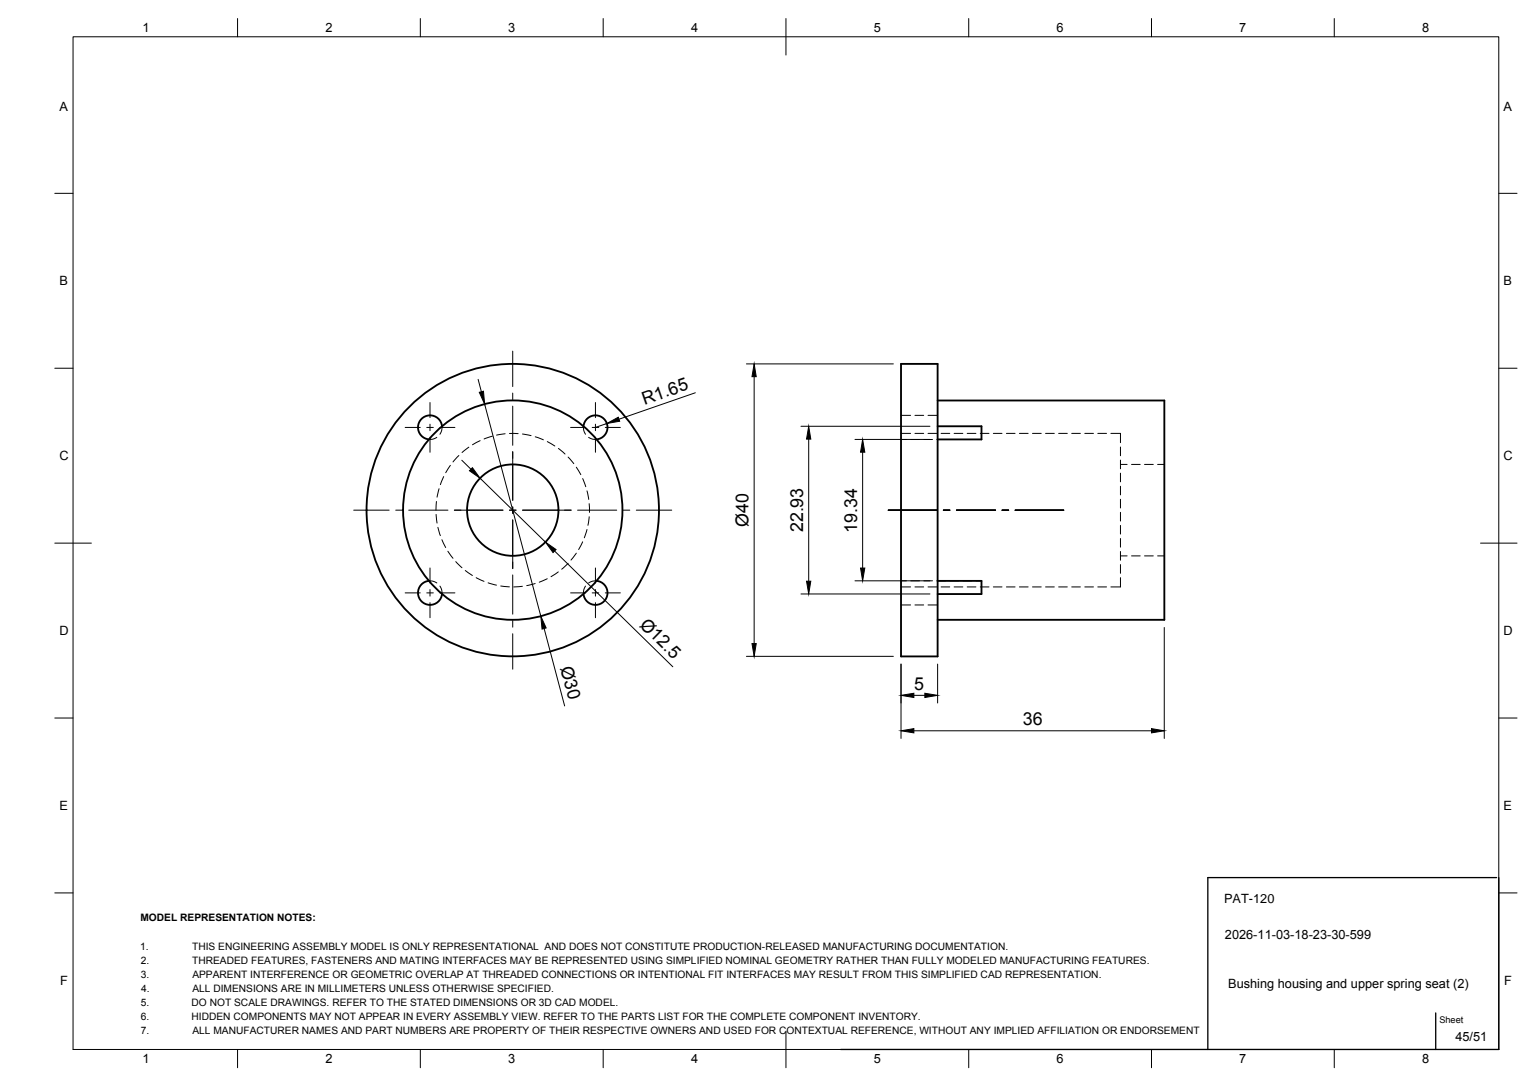
ISO-10303-21;
HEADER;
/* Generated by software containing ST-Developer
 * from STEP Tools, Inc. (www.steptools.com) 
 */

FILE_DESCRIPTION(
/* description */ ('Vibration shaker table dummy'),
/* implementation_level */ '2;1');

FILE_NAME(
/* name */ 'Bushing housing and upper spring seat (2).step',
/* time_stamp */ '2026-10-27T10:55:14-07:00',
/* author */ (''),
/* organization */ (''),
/* preprocessor_version */ 'ST-DEVELOPER v20.2',
/* originating_system */ 'Autodesk Translation Framework v15.17.0.0',
/* authorisation */ '');

FILE_SCHEMA (('AUTOMOTIVE_DESIGN { 1 0 10303 214 3 1 1 }'));
ENDSEC;

DATA;
#10=MECHANICAL_DESIGN_GEOMETRIC_PRESENTATION_REPRESENTATION('',(#726),#22394);
#634=SHAPE_REPRESENTATION_RELATIONSHIP('SRR','None',#22681,#680);
#680=ADVANCED_BREP_SHAPE_REPRESENTATION('',(#770),#22387);
#726=STYLED_ITEM('',(#22961),#770);
#770=MANIFOLD_SOLID_BREP('Body1',#9246);
#1023=FACE_BOUND('',#2513,.T.);
#1024=FACE_BOUND('',#2515,.T.);
#1025=FACE_BOUND('',#2519,.T.);
#1026=FACE_BOUND('',#2520,.T.);
#1027=FACE_BOUND('',#2521,.T.);
#1028=FACE_BOUND('',#2522,.T.);
#1029=FACE_BOUND('',#2523,.T.);
#1030=FACE_BOUND('',#2525,.T.);
#1294=PLANE('',#10616);
#1295=PLANE('',#10623);
#1296=PLANE('',#10630);
#1297=PLANE('',#10637);
#1298=PLANE('',#10654);
#1299=PLANE('',#10656);
#1300=PLANE('',#10662);
#1301=PLANE('',#10663);
#1756=FACE_OUTER_BOUND('',#2502,.T.);
#1757=FACE_OUTER_BOUND('',#2503,.T.);
#1758=FACE_OUTER_BOUND('',#2504,.T.);
#1759=FACE_OUTER_BOUND('',#2505,.T.);
#1760=FACE_OUTER_BOUND('',#2506,.T.);
#1761=FACE_OUTER_BOUND('',#2507,.T.);
#1762=FACE_OUTER_BOUND('',#2508,.T.);
#1763=FACE_OUTER_BOUND('',#2509,.T.);
#1764=FACE_OUTER_BOUND('',#2510,.T.);
#1765=FACE_OUTER_BOUND('',#2511,.T.);
#1766=FACE_OUTER_BOUND('',#2512,.T.);
#1767=FACE_OUTER_BOUND('',#2514,.T.);
#1768=FACE_OUTER_BOUND('',#2516,.T.);
#1769=FACE_OUTER_BOUND('',#2517,.T.);
#1770=FACE_OUTER_BOUND('',#2518,.T.);
#1771=FACE_OUTER_BOUND('',#2524,.T.);
#2502=EDGE_LOOP('',(#8118,#8119));
#2503=EDGE_LOOP('',(#8120,#8121,#8122,#8123,#8124,#8125,#8126,#8127));
#2504=EDGE_LOOP('',(#8128,#8129));
#2505=EDGE_LOOP('',(#8130,#8131,#8132,#8133,#8134,#8135,#8136,#8137));
#2506=EDGE_LOOP('',(#8138,#8139,#8140));
#2507=EDGE_LOOP('',(#8141,#8142,#8143,#8144,#8145,#8146,#8147,#8148));
#2508=EDGE_LOOP('',(#8149,#8150,#8151));
#2509=EDGE_LOOP('',(#8152,#8153,#8154,#8155,#8156,#8157,#8158,#8159));
#2510=EDGE_LOOP('',(#8160,#8161,#8162,#8163,#8164,#8165,#8166,#8167,#8168,
#8169,#8170,#8171,#8172,#8173,#8174,#8175,#8176,#8177,#8178,#8179));
#2511=EDGE_LOOP('',(#8180,#8181,#8182,#8183));
#2512=EDGE_LOOP('',(#8184));
#2513=EDGE_LOOP('',(#8185));
#2514=EDGE_LOOP('',(#8186));
#2515=EDGE_LOOP('',(#8187,#8188,#8189,#8190,#8191,#8192,#8193,#8194,#8195,
#8196,#8197));
#2516=EDGE_LOOP('',(#8198,#8199,#8200,#8201));
#2517=EDGE_LOOP('',(#8202,#8203,#8204,#8205));
#2518=EDGE_LOOP('',(#8206));
#2519=EDGE_LOOP('',(#8207));
#2520=EDGE_LOOP('',(#8208));
#2521=EDGE_LOOP('',(#8209));
#2522=EDGE_LOOP('',(#8210));
#2523=EDGE_LOOP('',(#8211));
#2524=EDGE_LOOP('',(#8212));
#2525=EDGE_LOOP('',(#8213));
#3153=LINE('',#21750,#3772);
#3154=LINE('',#21754,#3773);
#3155=LINE('',#21758,#3774);
#3156=LINE('',#21766,#3775);
#3157=LINE('',#21770,#3776);
#3158=LINE('',#21774,#3777);
#3159=LINE('',#21784,#3778);
#3160=LINE('',#21787,#3779);
#3161=LINE('',#21789,#3780);
#3162=LINE('',#21800,#3781);
#3163=LINE('',#21803,#3782);
#3164=LINE('',#21805,#3783);
#3165=LINE('',#21811,#3784);
#3166=LINE('',#21821,#3785);
#3167=LINE('',#21832,#3786);
#3168=LINE('',#21835,#3787);
#3772=VECTOR('',#13201,1.);
#3773=VECTOR('',#13204,0.165);
#3774=VECTOR('',#13209,1.);
#3775=VECTOR('',#13218,1.);
#3776=VECTOR('',#13221,0.165);
#3777=VECTOR('',#13226,1.);
#3778=VECTOR('',#13237,1.);
#3779=VECTOR('',#13240,1.);
#3780=VECTOR('',#13241,0.165);
#3781=VECTOR('',#13254,1.);
#3782=VECTOR('',#13257,1.);
#3783=VECTOR('',#13258,0.165);
#3784=VECTOR('',#13265,1.5);
#3785=VECTOR('',#13280,1.05);
#3786=VECTOR('',#13295,2.);
#3787=VECTOR('',#13298,0.625);
#4261=CIRCLE('',#10617,1.5);
#4262=CIRCLE('',#10618,0.165);
#4263=CIRCLE('',#10620,0.165);
#4264=CIRCLE('',#10621,0.165);
#4265=CIRCLE('',#10622,0.165);
#4266=CIRCLE('',#10624,1.5);
#4267=CIRCLE('',#10625,0.165);
#4268=CIRCLE('',#10627,0.165);
#4269=CIRCLE('',#10628,0.165);
#4270=CIRCLE('',#10629,0.165);
#4271=CIRCLE('',#10631,1.5);
#4272=CIRCLE('',#10632,0.165);
#4273=CIRCLE('',#10633,0.165);
#4274=CIRCLE('',#10635,0.165);
#4275=CIRCLE('',#10636,0.165);
#4276=CIRCLE('',#10638,1.5);
#4277=CIRCLE('',#10639,0.165);
#4278=CIRCLE('',#10640,0.165);
#4279=CIRCLE('',#10642,0.165);
#4280=CIRCLE('',#10643,0.165);
#4281=CIRCLE('',#10645,1.5);
#4282=CIRCLE('',#10646,1.5);
#4283=CIRCLE('',#10647,1.5);
#4284=CIRCLE('',#10648,1.5);
#4285=CIRCLE('',#10649,1.5);
#4286=CIRCLE('',#10650,1.5);
#4287=CIRCLE('',#10652,1.05);
#4288=CIRCLE('',#10653,1.05);
#4289=CIRCLE('',#10655,0.625);
#4290=CIRCLE('',#10657,2.);
#4291=CIRCLE('',#10659,2.);
#4292=CIRCLE('',#10661,0.625);
#4988=VERTEX_POINT('',#21744);
#4989=VERTEX_POINT('',#21745);
#4990=VERTEX_POINT('',#21749);
#4991=VERTEX_POINT('',#21751);
#4992=VERTEX_POINT('',#21753);
#4993=VERTEX_POINT('',#21756);
#4994=VERTEX_POINT('',#21760);
#4995=VERTEX_POINT('',#21761);
#4996=VERTEX_POINT('',#21765);
#4997=VERTEX_POINT('',#21767);
#4998=VERTEX_POINT('',#21769);
#4999=VERTEX_POINT('',#21772);
#5000=VERTEX_POINT('',#21776);
#5001=VERTEX_POINT('',#21777);
#5002=VERTEX_POINT('',#21779);
#5003=VERTEX_POINT('',#21783);
#5004=VERTEX_POINT('',#21785);
#5005=VERTEX_POINT('',#21788);
#5006=VERTEX_POINT('',#21792);
#5007=VERTEX_POINT('',#21793);
#5008=VERTEX_POINT('',#21795);
#5009=VERTEX_POINT('',#21799);
#5010=VERTEX_POINT('',#21801);
#5011=VERTEX_POINT('',#21804);
#5012=VERTEX_POINT('',#21808);
#5013=VERTEX_POINT('',#21810);
#5014=VERTEX_POINT('',#21818);
#5015=VERTEX_POINT('',#21820);
#5016=VERTEX_POINT('',#21824);
#5017=VERTEX_POINT('',#21827);
#5018=VERTEX_POINT('',#21830);
#5019=VERTEX_POINT('',#21834);
#6052=EDGE_CURVE('',#4988,#4989,#4261,.T.);
#6053=EDGE_CURVE('',#4988,#4989,#4262,.T.);
#6054=EDGE_CURVE('',#4990,#4988,#3153,.T.);
#6055=EDGE_CURVE('',#4991,#4990,#4263,.T.);
#6056=EDGE_CURVE('',#4991,#4992,#3154,.T.);
#6057=EDGE_CURVE('',#4992,#4992,#4264,.T.);
#6058=EDGE_CURVE('',#4993,#4991,#4265,.T.);
#6059=EDGE_CURVE('',#4989,#4993,#3155,.T.);
#6060=EDGE_CURVE('',#4994,#4995,#4266,.T.);
#6061=EDGE_CURVE('',#4994,#4995,#4267,.T.);
#6062=EDGE_CURVE('',#4996,#4994,#3156,.T.);
#6063=EDGE_CURVE('',#4997,#4996,#4268,.T.);
#6064=EDGE_CURVE('',#4997,#4998,#3157,.T.);
#6065=EDGE_CURVE('',#4998,#4998,#4269,.T.);
#6066=EDGE_CURVE('',#4999,#4997,#4270,.T.);
#6067=EDGE_CURVE('',#4995,#4999,#3158,.T.);
#6068=EDGE_CURVE('',#5000,#5001,#4271,.T.);
#6069=EDGE_CURVE('',#5000,#5002,#4272,.T.);
#6070=EDGE_CURVE('',#5002,#5001,#4273,.T.);
#6071=EDGE_CURVE('',#5003,#5000,#3159,.T.);
#6072=EDGE_CURVE('',#5004,#5003,#4274,.T.);
#6073=EDGE_CURVE('',#5001,#5004,#3160,.T.);
#6074=EDGE_CURVE('',#5002,#5005,#3161,.T.);
#6075=EDGE_CURVE('',#5005,#5005,#4275,.T.);
#6076=EDGE_CURVE('',#5006,#5007,#4276,.T.);
#6077=EDGE_CURVE('',#5006,#5008,#4277,.T.);
#6078=EDGE_CURVE('',#5008,#5007,#4278,.T.);
#6079=EDGE_CURVE('',#5009,#5006,#3162,.T.);
#6080=EDGE_CURVE('',#5010,#5009,#4279,.T.);
#6081=EDGE_CURVE('',#5007,#5010,#3163,.T.);
#6082=EDGE_CURVE('',#5008,#5011,#3164,.T.);
#6083=EDGE_CURVE('',#5011,#5011,#4280,.T.);
#6084=EDGE_CURVE('',#4993,#5012,#4281,.T.);
#6085=EDGE_CURVE('',#5012,#5013,#3165,.T.);
#6086=EDGE_CURVE('',#5013,#5013,#4282,.T.);
#6087=EDGE_CURVE('',#5012,#4996,#4283,.T.);
#6088=EDGE_CURVE('',#4999,#5003,#4284,.T.);
#6089=EDGE_CURVE('',#5004,#5009,#4285,.T.);
#6090=EDGE_CURVE('',#5010,#4990,#4286,.T.);
#6091=EDGE_CURVE('',#5014,#5014,#4287,.T.);
#6092=EDGE_CURVE('',#5014,#5015,#3166,.T.);
#6093=EDGE_CURVE('',#5015,#5015,#4288,.T.);
#6094=EDGE_CURVE('',#5016,#5016,#4289,.T.);
#6095=EDGE_CURVE('',#5017,#5017,#4290,.T.);
#6096=EDGE_CURVE('',#5018,#5018,#4291,.T.);
#6097=EDGE_CURVE('',#5018,#5017,#3167,.T.);
#6098=EDGE_CURVE('',#5016,#5019,#3168,.T.);
#6099=EDGE_CURVE('',#5019,#5019,#4292,.T.);
#8118=ORIENTED_EDGE('',*,*,#6052,.F.);
#8119=ORIENTED_EDGE('',*,*,#6053,.T.);
#8120=ORIENTED_EDGE('',*,*,#6054,.F.);
#8121=ORIENTED_EDGE('',*,*,#6055,.F.);
#8122=ORIENTED_EDGE('',*,*,#6056,.T.);
#8123=ORIENTED_EDGE('',*,*,#6057,.F.);
#8124=ORIENTED_EDGE('',*,*,#6056,.F.);
#8125=ORIENTED_EDGE('',*,*,#6058,.F.);
#8126=ORIENTED_EDGE('',*,*,#6059,.F.);
#8127=ORIENTED_EDGE('',*,*,#6053,.F.);
#8128=ORIENTED_EDGE('',*,*,#6060,.F.);
#8129=ORIENTED_EDGE('',*,*,#6061,.T.);
#8130=ORIENTED_EDGE('',*,*,#6062,.F.);
#8131=ORIENTED_EDGE('',*,*,#6063,.F.);
#8132=ORIENTED_EDGE('',*,*,#6064,.T.);
#8133=ORIENTED_EDGE('',*,*,#6065,.F.);
#8134=ORIENTED_EDGE('',*,*,#6064,.F.);
#8135=ORIENTED_EDGE('',*,*,#6066,.F.);
#8136=ORIENTED_EDGE('',*,*,#6067,.F.);
#8137=ORIENTED_EDGE('',*,*,#6061,.F.);
#8138=ORIENTED_EDGE('',*,*,#6068,.F.);
#8139=ORIENTED_EDGE('',*,*,#6069,.T.);
#8140=ORIENTED_EDGE('',*,*,#6070,.T.);
#8141=ORIENTED_EDGE('',*,*,#6071,.F.);
#8142=ORIENTED_EDGE('',*,*,#6072,.F.);
#8143=ORIENTED_EDGE('',*,*,#6073,.F.);
#8144=ORIENTED_EDGE('',*,*,#6070,.F.);
#8145=ORIENTED_EDGE('',*,*,#6074,.T.);
#8146=ORIENTED_EDGE('',*,*,#6075,.F.);
#8147=ORIENTED_EDGE('',*,*,#6074,.F.);
#8148=ORIENTED_EDGE('',*,*,#6069,.F.);
#8149=ORIENTED_EDGE('',*,*,#6076,.F.);
#8150=ORIENTED_EDGE('',*,*,#6077,.T.);
#8151=ORIENTED_EDGE('',*,*,#6078,.T.);
#8152=ORIENTED_EDGE('',*,*,#6079,.F.);
#8153=ORIENTED_EDGE('',*,*,#6080,.F.);
#8154=ORIENTED_EDGE('',*,*,#6081,.F.);
#8155=ORIENTED_EDGE('',*,*,#6078,.F.);
#8156=ORIENTED_EDGE('',*,*,#6082,.T.);
#8157=ORIENTED_EDGE('',*,*,#6083,.F.);
#8158=ORIENTED_EDGE('',*,*,#6082,.F.);
#8159=ORIENTED_EDGE('',*,*,#6077,.F.);
#8160=ORIENTED_EDGE('',*,*,#6054,.T.);
#8161=ORIENTED_EDGE('',*,*,#6052,.T.);
#8162=ORIENTED_EDGE('',*,*,#6059,.T.);
#8163=ORIENTED_EDGE('',*,*,#6084,.T.);
#8164=ORIENTED_EDGE('',*,*,#6085,.T.);
#8165=ORIENTED_EDGE('',*,*,#6086,.T.);
#8166=ORIENTED_EDGE('',*,*,#6085,.F.);
#8167=ORIENTED_EDGE('',*,*,#6087,.T.);
#8168=ORIENTED_EDGE('',*,*,#6062,.T.);
#8169=ORIENTED_EDGE('',*,*,#6060,.T.);
#8170=ORIENTED_EDGE('',*,*,#6067,.T.);
#8171=ORIENTED_EDGE('',*,*,#6088,.T.);
#8172=ORIENTED_EDGE('',*,*,#6071,.T.);
#8173=ORIENTED_EDGE('',*,*,#6068,.T.);
#8174=ORIENTED_EDGE('',*,*,#6073,.T.);
#8175=ORIENTED_EDGE('',*,*,#6089,.T.);
#8176=ORIENTED_EDGE('',*,*,#6079,.T.);
#8177=ORIENTED_EDGE('',*,*,#6076,.T.);
#8178=ORIENTED_EDGE('',*,*,#6081,.T.);
#8179=ORIENTED_EDGE('',*,*,#6090,.T.);
#8180=ORIENTED_EDGE('',*,*,#6091,.F.);
#8181=ORIENTED_EDGE('',*,*,#6092,.T.);
#8182=ORIENTED_EDGE('',*,*,#6093,.F.);
#8183=ORIENTED_EDGE('',*,*,#6092,.F.);
#8184=ORIENTED_EDGE('',*,*,#6091,.T.);
#8185=ORIENTED_EDGE('',*,*,#6094,.F.);
#8186=ORIENTED_EDGE('',*,*,#6095,.F.);
#8187=ORIENTED_EDGE('',*,*,#6058,.T.);
#8188=ORIENTED_EDGE('',*,*,#6055,.T.);
#8189=ORIENTED_EDGE('',*,*,#6090,.F.);
#8190=ORIENTED_EDGE('',*,*,#6080,.T.);
#8191=ORIENTED_EDGE('',*,*,#6089,.F.);
#8192=ORIENTED_EDGE('',*,*,#6072,.T.);
#8193=ORIENTED_EDGE('',*,*,#6088,.F.);
#8194=ORIENTED_EDGE('',*,*,#6066,.T.);
#8195=ORIENTED_EDGE('',*,*,#6063,.T.);
#8196=ORIENTED_EDGE('',*,*,#6087,.F.);
#8197=ORIENTED_EDGE('',*,*,#6084,.F.);
#8198=ORIENTED_EDGE('',*,*,#6096,.F.);
#8199=ORIENTED_EDGE('',*,*,#6097,.T.);
#8200=ORIENTED_EDGE('',*,*,#6095,.T.);
#8201=ORIENTED_EDGE('',*,*,#6097,.F.);
#8202=ORIENTED_EDGE('',*,*,#6094,.T.);
#8203=ORIENTED_EDGE('',*,*,#6098,.T.);
#8204=ORIENTED_EDGE('',*,*,#6099,.T.);
#8205=ORIENTED_EDGE('',*,*,#6098,.F.);
#8206=ORIENTED_EDGE('',*,*,#6096,.T.);
#8207=ORIENTED_EDGE('',*,*,#6093,.T.);
#8208=ORIENTED_EDGE('',*,*,#6083,.T.);
#8209=ORIENTED_EDGE('',*,*,#6075,.T.);
#8210=ORIENTED_EDGE('',*,*,#6065,.T.);
#8211=ORIENTED_EDGE('',*,*,#6057,.T.);
#8212=ORIENTED_EDGE('',*,*,#6086,.F.);
#8213=ORIENTED_EDGE('',*,*,#6099,.F.);
#8674=CYLINDRICAL_SURFACE('',#10619,0.165);
#8675=CYLINDRICAL_SURFACE('',#10626,0.165);
#8676=CYLINDRICAL_SURFACE('',#10634,0.165);
#8677=CYLINDRICAL_SURFACE('',#10641,0.165);
#8678=CYLINDRICAL_SURFACE('',#10644,1.5);
#8679=CYLINDRICAL_SURFACE('',#10651,1.05);
#8680=CYLINDRICAL_SURFACE('',#10658,2.);
#8681=CYLINDRICAL_SURFACE('',#10660,0.625);
#9121=ADVANCED_FACE('',(#1756),#1294,.T.);
#9122=ADVANCED_FACE('',(#1757),#8674,.F.);
#9123=ADVANCED_FACE('',(#1758),#1295,.T.);
#9124=ADVANCED_FACE('',(#1759),#8675,.F.);
#9125=ADVANCED_FACE('',(#1760),#1296,.T.);
#9126=ADVANCED_FACE('',(#1761),#8676,.F.);
#9127=ADVANCED_FACE('',(#1762),#1297,.T.);
#9128=ADVANCED_FACE('',(#1763),#8677,.F.);
#9129=ADVANCED_FACE('',(#1764),#8678,.T.);
#9130=ADVANCED_FACE('',(#1765),#8679,.F.);
#9131=ADVANCED_FACE('',(#1766,#1023),#1298,.T.);
#9132=ADVANCED_FACE('',(#1767,#1024),#1299,.F.);
#9133=ADVANCED_FACE('',(#1768),#8680,.T.);
#9134=ADVANCED_FACE('',(#1769),#8681,.F.);
#9135=ADVANCED_FACE('',(#1770,#1025,#1026,#1027,#1028,#1029),#1300,.T.);
#9136=ADVANCED_FACE('',(#1771,#1030),#1301,.F.);
#9246=CLOSED_SHELL('',(#9121,#9122,#9123,#9124,#9125,#9126,#9127,#9128,
#9129,#9130,#9131,#9132,#9133,#9134,#9135,#9136));
#10615=AXIS2_PLACEMENT_3D('',#21742,#13191,#13192);
#10616=AXIS2_PLACEMENT_3D('',#21743,#13193,#13194);
#10617=AXIS2_PLACEMENT_3D('',#21746,#13195,#13196);
#10618=AXIS2_PLACEMENT_3D('',#21747,#13197,#13198);
#10619=AXIS2_PLACEMENT_3D('',#21748,#13199,#13200);
#10620=AXIS2_PLACEMENT_3D('',#21752,#13202,#13203);
#10621=AXIS2_PLACEMENT_3D('',#21755,#13205,#13206);
#10622=AXIS2_PLACEMENT_3D('',#21757,#13207,#13208);
#10623=AXIS2_PLACEMENT_3D('',#21759,#13210,#13211);
#10624=AXIS2_PLACEMENT_3D('',#21762,#13212,#13213);
#10625=AXIS2_PLACEMENT_3D('',#21763,#13214,#13215);
#10626=AXIS2_PLACEMENT_3D('',#21764,#13216,#13217);
#10627=AXIS2_PLACEMENT_3D('',#21768,#13219,#13220);
#10628=AXIS2_PLACEMENT_3D('',#21771,#13222,#13223);
#10629=AXIS2_PLACEMENT_3D('',#21773,#13224,#13225);
#10630=AXIS2_PLACEMENT_3D('',#21775,#13227,#13228);
#10631=AXIS2_PLACEMENT_3D('',#21778,#13229,#13230);
#10632=AXIS2_PLACEMENT_3D('',#21780,#13231,#13232);
#10633=AXIS2_PLACEMENT_3D('',#21781,#13233,#13234);
#10634=AXIS2_PLACEMENT_3D('',#21782,#13235,#13236);
#10635=AXIS2_PLACEMENT_3D('',#21786,#13238,#13239);
#10636=AXIS2_PLACEMENT_3D('',#21790,#13242,#13243);
#10637=AXIS2_PLACEMENT_3D('',#21791,#13244,#13245);
#10638=AXIS2_PLACEMENT_3D('',#21794,#13246,#13247);
#10639=AXIS2_PLACEMENT_3D('',#21796,#13248,#13249);
#10640=AXIS2_PLACEMENT_3D('',#21797,#13250,#13251);
#10641=AXIS2_PLACEMENT_3D('',#21798,#13252,#13253);
#10642=AXIS2_PLACEMENT_3D('',#21802,#13255,#13256);
#10643=AXIS2_PLACEMENT_3D('',#21806,#13259,#13260);
#10644=AXIS2_PLACEMENT_3D('',#21807,#13261,#13262);
#10645=AXIS2_PLACEMENT_3D('',#21809,#13263,#13264);
#10646=AXIS2_PLACEMENT_3D('',#21812,#13266,#13267);
#10647=AXIS2_PLACEMENT_3D('',#21813,#13268,#13269);
#10648=AXIS2_PLACEMENT_3D('',#21814,#13270,#13271);
#10649=AXIS2_PLACEMENT_3D('',#21815,#13272,#13273);
#10650=AXIS2_PLACEMENT_3D('',#21816,#13274,#13275);
#10651=AXIS2_PLACEMENT_3D('',#21817,#13276,#13277);
#10652=AXIS2_PLACEMENT_3D('',#21819,#13278,#13279);
#10653=AXIS2_PLACEMENT_3D('',#21822,#13281,#13282);
#10654=AXIS2_PLACEMENT_3D('',#21823,#13283,#13284);
#10655=AXIS2_PLACEMENT_3D('',#21825,#13285,#13286);
#10656=AXIS2_PLACEMENT_3D('',#21826,#13287,#13288);
#10657=AXIS2_PLACEMENT_3D('',#21828,#13289,#13290);
#10658=AXIS2_PLACEMENT_3D('',#21829,#13291,#13292);
#10659=AXIS2_PLACEMENT_3D('',#21831,#13293,#13294);
#10660=AXIS2_PLACEMENT_3D('',#21833,#13296,#13297);
#10661=AXIS2_PLACEMENT_3D('',#21836,#13299,#13300);
#10662=AXIS2_PLACEMENT_3D('',#21837,#13301,#13302);
#10663=AXIS2_PLACEMENT_3D('',#21838,#13303,#13304);
#13191=DIRECTION('axis',(0.,0.,1.));
#13192=DIRECTION('refdir',(1.,0.,0.));
#13193=DIRECTION('center_axis',(0.,0.,1.));
#13194=DIRECTION('ref_axis',(1.,0.,0.));
#13195=DIRECTION('center_axis',(0.,0.,-1.));
#13196=DIRECTION('ref_axis',(1.,0.,0.));
#13197=DIRECTION('center_axis',(0.,0.,1.));
#13198=DIRECTION('ref_axis',(1.,0.,0.));
#13199=DIRECTION('center_axis',(0.,0.,1.));
#13200=DIRECTION('ref_axis',(1.,0.,0.));
#13201=DIRECTION('',(0.,0.,-1.));
#13202=DIRECTION('center_axis',(0.,0.,1.));
#13203=DIRECTION('ref_axis',(1.,0.,0.));
#13204=DIRECTION('',(0.,0.,1.));
#13205=DIRECTION('center_axis',(0.,0.,-1.));
#13206=DIRECTION('ref_axis',(1.,0.,0.));
#13207=DIRECTION('center_axis',(0.,0.,1.));
#13208=DIRECTION('ref_axis',(1.,0.,0.));
#13209=DIRECTION('',(0.,0.,1.));
#13210=DIRECTION('center_axis',(0.,0.,1.));
#13211=DIRECTION('ref_axis',(1.,0.,0.));
#13212=DIRECTION('center_axis',(0.,0.,-1.));
#13213=DIRECTION('ref_axis',(1.,0.,0.));
#13214=DIRECTION('center_axis',(0.,0.,1.));
#13215=DIRECTION('ref_axis',(1.,0.,0.));
#13216=DIRECTION('center_axis',(0.,0.,1.));
#13217=DIRECTION('ref_axis',(1.,0.,0.));
#13218=DIRECTION('',(0.,0.,-1.));
#13219=DIRECTION('center_axis',(0.,0.,1.));
#13220=DIRECTION('ref_axis',(1.,0.,0.));
#13221=DIRECTION('',(0.,0.,1.));
#13222=DIRECTION('center_axis',(0.,0.,-1.));
#13223=DIRECTION('ref_axis',(1.,0.,0.));
#13224=DIRECTION('center_axis',(0.,0.,1.));
#13225=DIRECTION('ref_axis',(1.,0.,0.));
#13226=DIRECTION('',(0.,0.,1.));
#13227=DIRECTION('center_axis',(0.,0.,1.));
#13228=DIRECTION('ref_axis',(1.,0.,0.));
#13229=DIRECTION('center_axis',(0.,0.,-1.));
#13230=DIRECTION('ref_axis',(1.,0.,0.));
#13231=DIRECTION('center_axis',(0.,0.,1.));
#13232=DIRECTION('ref_axis',(1.,0.,0.));
#13233=DIRECTION('center_axis',(0.,0.,1.));
#13234=DIRECTION('ref_axis',(1.,0.,0.));
#13235=DIRECTION('center_axis',(0.,0.,1.));
#13236=DIRECTION('ref_axis',(1.,0.,0.));
#13237=DIRECTION('',(0.,0.,-1.));
#13238=DIRECTION('center_axis',(0.,0.,1.));
#13239=DIRECTION('ref_axis',(1.,0.,0.));
#13240=DIRECTION('',(0.,0.,1.));
#13241=DIRECTION('',(0.,0.,1.));
#13242=DIRECTION('center_axis',(0.,0.,-1.));
#13243=DIRECTION('ref_axis',(1.,0.,0.));
#13244=DIRECTION('center_axis',(0.,0.,1.));
#13245=DIRECTION('ref_axis',(1.,0.,0.));
#13246=DIRECTION('center_axis',(0.,0.,-1.));
#13247=DIRECTION('ref_axis',(1.,0.,0.));
#13248=DIRECTION('center_axis',(0.,0.,1.));
#13249=DIRECTION('ref_axis',(1.,0.,0.));
#13250=DIRECTION('center_axis',(0.,0.,1.));
#13251=DIRECTION('ref_axis',(1.,0.,0.));
#13252=DIRECTION('center_axis',(0.,0.,1.));
#13253=DIRECTION('ref_axis',(1.,0.,0.));
#13254=DIRECTION('',(0.,0.,-1.));
#13255=DIRECTION('center_axis',(0.,0.,1.));
#13256=DIRECTION('ref_axis',(1.,0.,0.));
#13257=DIRECTION('',(0.,0.,1.));
#13258=DIRECTION('',(0.,0.,1.));
#13259=DIRECTION('center_axis',(0.,0.,-1.));
#13260=DIRECTION('ref_axis',(1.,0.,0.));
#13261=DIRECTION('center_axis',(0.,0.,1.));
#13262=DIRECTION('ref_axis',(1.,0.,0.));
#13263=DIRECTION('center_axis',(0.,0.,-1.));
#13264=DIRECTION('ref_axis',(1.,0.,0.));
#13265=DIRECTION('',(0.,0.,-1.));
#13266=DIRECTION('center_axis',(0.,0.,1.));
#13267=DIRECTION('ref_axis',(1.,0.,0.));
#13268=DIRECTION('center_axis',(0.,0.,-1.));
#13269=DIRECTION('ref_axis',(1.,0.,0.));
#13270=DIRECTION('center_axis',(0.,0.,-1.));
#13271=DIRECTION('ref_axis',(1.,0.,0.));
#13272=DIRECTION('center_axis',(0.,0.,-1.));
#13273=DIRECTION('ref_axis',(1.,0.,0.));
#13274=DIRECTION('center_axis',(0.,0.,-1.));
#13275=DIRECTION('ref_axis',(1.,0.,0.));
#13276=DIRECTION('center_axis',(0.,0.,1.));
#13277=DIRECTION('ref_axis',(1.,0.,0.));
#13278=DIRECTION('center_axis',(0.,0.,1.));
#13279=DIRECTION('ref_axis',(1.,0.,0.));
#13280=DIRECTION('',(0.,0.,1.));
#13281=DIRECTION('center_axis',(0.,0.,-1.));
#13282=DIRECTION('ref_axis',(1.,0.,0.));
#13283=DIRECTION('center_axis',(0.,0.,1.));
#13284=DIRECTION('ref_axis',(1.,0.,0.));
#13285=DIRECTION('center_axis',(0.,0.,1.));
#13286=DIRECTION('ref_axis',(1.,0.,0.));
#13287=DIRECTION('center_axis',(0.,0.,1.));
#13288=DIRECTION('ref_axis',(1.,0.,0.));
#13289=DIRECTION('center_axis',(0.,0.,1.));
#13290=DIRECTION('ref_axis',(1.,0.,0.));
#13291=DIRECTION('center_axis',(0.,0.,1.));
#13292=DIRECTION('ref_axis',(1.,0.,0.));
#13293=DIRECTION('center_axis',(0.,0.,1.));
#13294=DIRECTION('ref_axis',(1.,0.,0.));
#13295=DIRECTION('',(0.,0.,-1.));
#13296=DIRECTION('center_axis',(0.,0.,1.));
#13297=DIRECTION('ref_axis',(1.,0.,0.));
#13298=DIRECTION('',(0.,0.,-1.));
#13299=DIRECTION('center_axis',(0.,0.,-1.));
#13300=DIRECTION('ref_axis',(1.,0.,0.));
#13301=DIRECTION('center_axis',(0.,0.,1.));
#13302=DIRECTION('ref_axis',(1.,0.,0.));
#13303=DIRECTION('center_axis',(0.,0.,1.));
#13304=DIRECTION('ref_axis',(1.,0.,0.));
#21742=CARTESIAN_POINT('',(0.,0.,0.));
#21743=CARTESIAN_POINT('Origin',(4.86862915010152,-5.13137084989848,14.));
#21744=CARTESIAN_POINT('',(5.03292205834015,-5.14662995545858,14.));
#21745=CARTESIAN_POINT('',(4.85337004454142,-4.96707794165985,14.));
#21746=CARTESIAN_POINT('Origin',(6.,-4.,14.));
#21747=CARTESIAN_POINT('Origin',(4.86862915010152,-5.13137084989848,14.));
#21748=CARTESIAN_POINT('Origin',(4.86862915010152,-5.13137084989848,14.));
#21749=CARTESIAN_POINT('',(5.03292205834015,-5.14662995545858,14.6));
#21750=CARTESIAN_POINT('',(5.03292205834015,-5.14662995545858,14.));
#21751=CARTESIAN_POINT('',(4.70362915010152,-5.13137084989848,14.6));
#21752=CARTESIAN_POINT('Origin',(4.86862915010152,-5.13137084989848,14.6));
#21753=CARTESIAN_POINT('',(4.70362915010152,-5.13137084989848,15.1));
#21754=CARTESIAN_POINT('',(4.70362915010152,-5.13137084989848,14.));
#21755=CARTESIAN_POINT('Origin',(4.86862915010152,-5.13137084989848,15.1));
#21756=CARTESIAN_POINT('',(4.85337004454142,-4.96707794165985,14.6));
#21757=CARTESIAN_POINT('Origin',(4.86862915010152,-5.13137084989848,14.6));
#21758=CARTESIAN_POINT('',(4.85337004454142,-4.96707794165985,14.));
#21759=CARTESIAN_POINT('Origin',(4.86862915010152,-2.86862915010152,14.));
#21760=CARTESIAN_POINT('',(4.85337004454142,-3.03292205834015,14.));
#21761=CARTESIAN_POINT('',(5.03292205834015,-2.85337004454142,14.));
#21762=CARTESIAN_POINT('Origin',(6.,-4.,14.));
#21763=CARTESIAN_POINT('Origin',(4.86862915010152,-2.86862915010152,14.));
#21764=CARTESIAN_POINT('Origin',(4.86862915010152,-2.86862915010152,14.));
#21765=CARTESIAN_POINT('',(4.85337004454142,-3.03292205834015,14.6));
#21766=CARTESIAN_POINT('',(4.85337004454142,-3.03292205834015,14.));
#21767=CARTESIAN_POINT('',(4.70362915010152,-2.86862915010152,14.6));
#21768=CARTESIAN_POINT('Origin',(4.86862915010152,-2.86862915010152,14.6));
#21769=CARTESIAN_POINT('',(4.70362915010152,-2.86862915010152,15.1));
#21770=CARTESIAN_POINT('',(4.70362915010152,-2.86862915010152,14.));
#21771=CARTESIAN_POINT('Origin',(4.86862915010152,-2.86862915010152,15.1));
#21772=CARTESIAN_POINT('',(5.03292205834015,-2.85337004454142,14.6));
#21773=CARTESIAN_POINT('Origin',(4.86862915010152,-2.86862915010152,14.6));
#21774=CARTESIAN_POINT('',(5.03292205834015,-2.85337004454142,14.));
#21775=CARTESIAN_POINT('Origin',(7.13137084989848,-2.86862915010152,14.));
#21776=CARTESIAN_POINT('',(6.96707794165985,-2.85337004454142,14.));
#21777=CARTESIAN_POINT('',(7.14662995545858,-3.03292205834015,14.));
#21778=CARTESIAN_POINT('Origin',(6.,-4.,14.));
#21779=CARTESIAN_POINT('',(6.96637084989848,-2.86862915010152,14.));
#21780=CARTESIAN_POINT('Origin',(7.13137084989848,-2.86862915010152,14.));
#21781=CARTESIAN_POINT('Origin',(7.13137084989848,-2.86862915010152,14.));
#21782=CARTESIAN_POINT('Origin',(7.13137084989848,-2.86862915010152,14.));
#21783=CARTESIAN_POINT('',(6.96707794165985,-2.85337004454142,14.6));
#21784=CARTESIAN_POINT('',(6.96707794165985,-2.85337004454142,14.));
#21785=CARTESIAN_POINT('',(7.14662995545858,-3.03292205834015,14.6));
#21786=CARTESIAN_POINT('Origin',(7.13137084989848,-2.86862915010152,14.6));
#21787=CARTESIAN_POINT('',(7.14662995545858,-3.03292205834015,14.));
#21788=CARTESIAN_POINT('',(6.96637084989848,-2.86862915010152,15.1));
#21789=CARTESIAN_POINT('',(6.96637084989848,-2.86862915010152,14.));
#21790=CARTESIAN_POINT('Origin',(7.13137084989848,-2.86862915010152,15.1));
#21791=CARTESIAN_POINT('Origin',(7.13137084989848,-5.13137084989848,14.));
#21792=CARTESIAN_POINT('',(7.14662995545858,-4.96707794165985,14.));
#21793=CARTESIAN_POINT('',(6.96707794165985,-5.14662995545858,14.));
#21794=CARTESIAN_POINT('Origin',(6.,-4.,14.));
#21795=CARTESIAN_POINT('',(6.96637084989848,-5.13137084989848,14.));
#21796=CARTESIAN_POINT('Origin',(7.13137084989848,-5.13137084989848,14.));
#21797=CARTESIAN_POINT('Origin',(7.13137084989848,-5.13137084989848,14.));
#21798=CARTESIAN_POINT('Origin',(7.13137084989848,-5.13137084989848,14.));
#21799=CARTESIAN_POINT('',(7.14662995545858,-4.96707794165985,14.6));
#21800=CARTESIAN_POINT('',(7.14662995545858,-4.96707794165985,14.));
#21801=CARTESIAN_POINT('',(6.96707794165985,-5.14662995545858,14.6));
#21802=CARTESIAN_POINT('Origin',(7.13137084989848,-5.13137084989848,14.6));
#21803=CARTESIAN_POINT('',(6.96707794165985,-5.14662995545858,14.));
#21804=CARTESIAN_POINT('',(6.96637084989848,-5.13137084989848,15.1));
#21805=CARTESIAN_POINT('',(6.96637084989848,-5.13137084989848,14.));
#21806=CARTESIAN_POINT('Origin',(7.13137084989848,-5.13137084989848,15.1));
#21807=CARTESIAN_POINT('Origin',(6.,-4.,11.5));
#21808=CARTESIAN_POINT('',(4.5,-4.,14.6));
#21809=CARTESIAN_POINT('Origin',(6.,-4.,14.6));
#21810=CARTESIAN_POINT('',(4.5,-4.,11.5));
#21811=CARTESIAN_POINT('',(4.5,-4.,11.5));
#21812=CARTESIAN_POINT('Origin',(6.,-4.,11.5));
#21813=CARTESIAN_POINT('Origin',(6.,-4.,14.6));
#21814=CARTESIAN_POINT('Origin',(6.,-4.,14.6));
#21815=CARTESIAN_POINT('Origin',(6.,-4.,14.6));
#21816=CARTESIAN_POINT('Origin',(6.,-4.,14.6));
#21817=CARTESIAN_POINT('Origin',(6.,-4.,12.1));
#21818=CARTESIAN_POINT('',(4.95,-4.,12.1));
#21819=CARTESIAN_POINT('Origin',(6.,-4.,12.1));
#21820=CARTESIAN_POINT('',(4.95,-4.,15.1));
#21821=CARTESIAN_POINT('',(4.95,-4.,12.1));
#21822=CARTESIAN_POINT('Origin',(6.,-4.,15.1));
#21823=CARTESIAN_POINT('Origin',(6.,-4.,12.1));
#21824=CARTESIAN_POINT('',(5.375,-4.,12.1));
#21825=CARTESIAN_POINT('Origin',(6.,-4.,12.1));
#21826=CARTESIAN_POINT('Origin',(6.,-4.,14.6));
#21827=CARTESIAN_POINT('',(4.,-4.,14.6));
#21828=CARTESIAN_POINT('Origin',(6.,-4.,14.6));
#21829=CARTESIAN_POINT('Origin',(6.,-4.,14.6));
#21830=CARTESIAN_POINT('',(4.,-4.,15.1));
#21831=CARTESIAN_POINT('Origin',(6.,-4.,15.1));
#21832=CARTESIAN_POINT('',(4.,-4.,14.6));
#21833=CARTESIAN_POINT('Origin',(6.,-4.,11.5));
#21834=CARTESIAN_POINT('',(5.375,-4.,11.5));
#21835=CARTESIAN_POINT('',(5.375,-4.,11.5));
#21836=CARTESIAN_POINT('Origin',(6.,-4.,11.5));
#21837=CARTESIAN_POINT('Origin',(6.,-4.,15.1));
#21838=CARTESIAN_POINT('Origin',(6.,-4.,11.5));
#22336=UNCERTAINTY_MEASURE_WITH_UNIT(LENGTH_MEASURE(0.001),#22395,
'DISTANCE_ACCURACY_VALUE',
'Maximum model space distance between geometric entities at asserted c
onnectivities');
#22343=UNCERTAINTY_MEASURE_WITH_UNIT(LENGTH_MEASURE(0.001),#22395,
'DISTANCE_ACCURACY_VALUE',
'Maximum model space distance between geometric entities at asserted c
onnectivities');
#22387=(
GEOMETRIC_REPRESENTATION_CONTEXT(3)
GLOBAL_UNCERTAINTY_ASSIGNED_CONTEXT((#22336))
GLOBAL_UNIT_ASSIGNED_CONTEXT((#22395,#22397,#22398))
REPRESENTATION_CONTEXT('','3D')
);
#22394=(
GEOMETRIC_REPRESENTATION_CONTEXT(3)
GLOBAL_UNCERTAINTY_ASSIGNED_CONTEXT((#22343))
GLOBAL_UNIT_ASSIGNED_CONTEXT((#22395,#22397,#22398))
REPRESENTATION_CONTEXT('','3D')
);
#22395=(
LENGTH_UNIT()
NAMED_UNIT(*)
SI_UNIT(.CENTI.,.METRE.)
);
#22397=(
NAMED_UNIT(*)
PLANE_ANGLE_UNIT()
SI_UNIT($,.RADIAN.)
);
#22398=(
NAMED_UNIT(*)
SI_UNIT($,.STERADIAN.)
SOLID_ANGLE_UNIT()
);
#22442=SHAPE_DEFINITION_REPRESENTATION(#22492,#22681);
#22492=PRODUCT_DEFINITION_SHAPE('',$,#22732);
#22681=SHAPE_REPRESENTATION('',(#10615),#22387);
#22688=PRODUCT_DEFINITION_CONTEXT('part definition',#22840,'design');
#22732=PRODUCT_DEFINITION('Bushing housing and upper spring seat (2)',
'Bushing housing and upper spring seat (2)',#22782,#22688);
#22782=PRODUCT_DEFINITION_FORMATION('',$,#22885);
#22840=APPLICATION_CONTEXT(
'Core Data for Automotive Mechanical Design Process');
#22841=PRODUCT_CONTEXT('part definition',#22840,'mechanical');
#22885=PRODUCT('Bushing housing and upper spring seat (2)',
'Bushing housing and upper spring seat (2)',
'Bushing housing and upper spring seat (2)',(#22841));
#22955=COLOUR_RGB('Grey',0.48,0.52,0.57);
#22956=FILL_AREA_STYLE_COLOUR('',#22955);
#22957=FILL_AREA_STYLE('',(#22956));
#22958=SURFACE_STYLE_FILL_AREA(#22957);
#22959=SURFACE_SIDE_STYLE('',(#22958));
#22960=SURFACE_STYLE_USAGE(.BOTH.,#22959);
#22961=PRESENTATION_STYLE_ASSIGNMENT((#22960));
ENDSEC;
END-ISO-10303-21;
